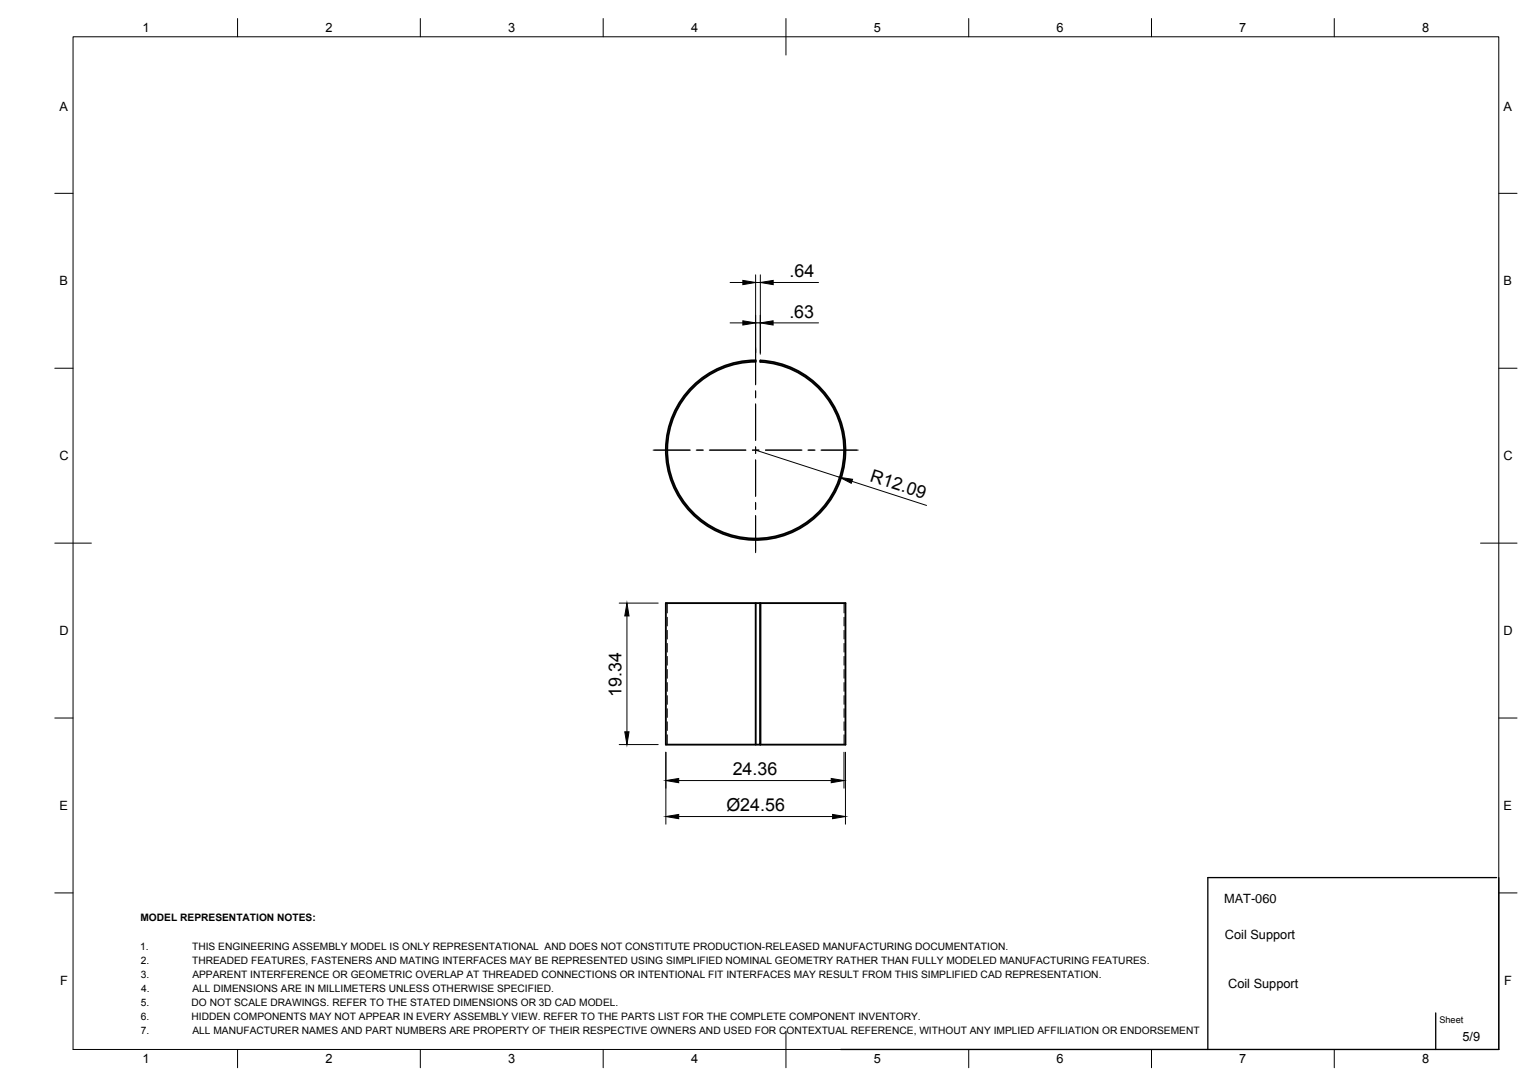
ISO-10303-21;
HEADER;
FILE_DESCRIPTION (('STEP AP214'),
    '1' );
FILE_NAME ('Coil Support.step',
    '2026-10-29T23:46:56',
    ( '' ),
    ( '' ),
    'SwSTEP 2.0',
    'SolidWorks 2020',
    '' );
FILE_SCHEMA (( 'AUTOMOTIVE_DESIGN' ));
ENDSEC;

DATA;
#93=APPLICATION_CONTEXT ( 'automotive_design' ) ;
#920=PLANE ( 'NONE',  #8989 ) ;
#938=UNCERTAINTY_MEASURE_WITH_UNIT (LENGTH_MEASURE( 1.000000000000000082E-05 ), #1682, 'distance_accuracy_value', 'NONE');
#1251=UNCERTAINTY_MEASURE_WITH_UNIT (LENGTH_MEASURE( 1.000000000000000082E-05 ), #14331, 'distance_accuracy_value', 'NONE');
#1354=DIRECTION ( 'NONE',  ( 0.000000000000000000, 0.000000000000000000, 1.000000000000000000 ) ) ;
#1682=( LENGTH_UNIT ( ) NAMED_UNIT ( * ) SI_UNIT ( .MILLI., .METRE. ) );
#1888=ADVANCED_FACE ( 'NONE', ( #14373 ), #14045, .F. ) ;
#2120=CIRCLE ( 'NONE', #12091, 12.08499999999999908 ) ;
#2336=DIRECTION ( 'NONE',  ( -1.000000000000000000, -6.722685822323786766E-17, 0.000000000000000000 ) ) ;
#2420=VECTOR ( 'NONE', #13652, 1000.000000000000000 ) ;
#2970=CARTESIAN_POINT ( 'NONE',  ( 8.823575513742490273, 15.24673779880127356, 47.37072134000479906 ) ) ;
#3223=FACE_OUTER_BOUND ( 'NONE', #6473, .T. ) ;
#3349=DIRECTION ( 'NONE',  ( -0.9996573249755574819, -1.344306794811909066E-16, 0.02617694830786587712 ) ) ;
#3732=ORIENTED_EDGE ( 'NONE', *, *, #20264, .T. ) ;
#3809=ADVANCED_FACE ( 'NONE', ( #18879 ), #11193, .T. ) ;
#3828=CARTESIAN_POINT ( 'NONE',  ( 8.823575513742486720, 34.59164230456639899, 47.37072134000479906 ) ) ;
#3965=EDGE_CURVE ( 'NONE', #14754, #4855, #5249, .T. ) ;
#4047=ORIENTED_EDGE ( 'NONE', *, *, #20264, .F. ) ;
#4080=CARTESIAN_POINT ( 'NONE',  ( 9.016997203727582288, 34.59164230456639899, 47.36565641480107303 ) ) ;
#4315=DIRECTION ( 'NONE',  ( -0.02617694830786587365, -1.759793992609925531E-18, 0.9996573249755574819 ) ) ;
#4409=ORIENTED_EDGE ( 'NONE', *, *, #26266, .F. ) ;
#4774=DIRECTION ( 'NONE',  ( -1.000000000000000000, 0.000000000000000000, 0.000000000000000000 ) ) ;
#4801=( NAMED_UNIT ( * ) SI_UNIT ( $, .STERADIAN. ) SOLID_ANGLE_UNIT ( ) );
#4810=CARTESIAN_POINT ( 'NONE',  ( 9.016997203727585841, 15.24673779880127356, 47.36565641480107303 ) ) ;
#4855=VERTEX_POINT ( 'NONE', #3828 ) ;
#4994=ORIENTED_EDGE ( 'NONE', *, *, #3965, .T. ) ;
#5249=LINE ( 'NONE', #15258, #5266 ) ;
#5266=VECTOR ( 'NONE', #25269, 1000.000000000000000 ) ;
#5378=CARTESIAN_POINT ( 'NONE',  ( 9.016997203727585841, 15.24673779880127356, 47.36565641480107303 ) ) ;
#5977=DIRECTION ( 'NONE',  ( 1.000000000000000000, 0.000000000000000000, 0.000000000000000000 ) ) ;
#6075=STYLED_ITEM ( 'NONE', ( #27283 ), #8502 ) ;
#6286=CARTESIAN_POINT ( 'NONE',  ( 0.000000000000000000, 0.000000000000000000, 0.000000000000000000 ) ) ;
#6354=ORIENTED_EDGE ( 'NONE', *, *, #20840, .T. ) ;
#6473=EDGE_LOOP ( 'NONE', ( #3732, #4994, #23188, #17455 ) ) ;
#6586=CARTESIAN_POINT ( 'NONE',  ( 21.09785597605719332, 34.59164230456639899, 47.04930799450051637 ) ) ;
#6613=( NAMED_UNIT ( * ) PLANE_ANGLE_UNIT ( ) SI_UNIT ( $, .RADIAN. ) );
#6740=VERTEX_POINT ( 'NONE', #4080 ) ;
#7156=PRODUCT_DEFINITION_CONTEXT ( 'detailed design', #29222, 'design' ) ;
#7164=ORIENTED_EDGE ( 'NONE', *, *, #11045, .F. ) ;
#7266=SURFACE_SIDE_STYLE ('',( #19066 ) ) ;
#7305=VERTEX_POINT ( 'NONE', #30199 ) ;
#8051=CARTESIAN_POINT ( 'NONE',  ( 9.016997203727585841, 15.24673779880127356, 46.73295957419995261 ) ) ;
#8162=DIRECTION ( 'NONE',  ( 0.02617694830786587712, 1.759793992609925531E-18, 0.9996573249755574819 ) ) ;
#8172=AXIS2_PLACEMENT_3D ( 'NONE', #6286, #1354, #5977 ) ;
#8284=CARTESIAN_POINT ( 'NONE',  ( 9.016997203727582288, 34.59164230456639899, 46.73295957419995261 ) ) ;
#8475=STYLED_ITEM('',(#32529),#12176);
#8502=ADVANCED_BREP_SHAPE_REPRESENTATION ( '', ( #12176, #8172 ), #26498 ) ;
#8989=AXIS2_PLACEMENT_3D ( 'NONE', #5378, #8162, #13260 ) ;
#9433=CARTESIAN_POINT ( 'NONE',  ( 8.823575513742490273, 15.24673779880127356, 47.37072134000479906 ) ) ;
#9482=ORIENTED_EDGE ( 'NONE', *, *, #11238, .T. ) ;
#9569=CARTESIAN_POINT ( 'NONE',  ( 9.016997203727585841, 15.24673779880127356, 46.73295957419995261 ) ) ;
#9604=ORIENTED_EDGE ( 'NONE', *, *, #19433, .F. ) ;
#9896=VECTOR ( 'NONE', #27905, 1000.000000000000000 ) ;
#10047=DIRECTION ( 'NONE',  ( -1.000000000000000000, 0.000000000000000000, 0.000000000000000000 ) ) ;
#10212=CARTESIAN_POINT ( 'NONE',  ( 9.016997203727582288, 34.59164230456639899, 46.73295957419995261 ) ) ;
#10249=ORIENTED_EDGE ( 'NONE', *, *, #26494, .F. ) ;
#10276=LINE ( 'NONE', #8284, #15201 ) ;
#10299=ORIENTED_EDGE ( 'NONE', *, *, #26494, .T. ) ;
#10924=CIRCLE ( 'NONE', #11970, 12.08499999999999552 ) ;
#11045=EDGE_CURVE ( 'NONE', #6740, #18267, #2120, .T. ) ;
#11193=CYLINDRICAL_SURFACE ( 'NONE', #18323, 12.27848799348799069 ) ;
#11238=EDGE_CURVE ( 'NONE', #14754, #7305, #26221, .T. ) ;
#11270=ORIENTED_EDGE ( 'NONE', *, *, #3965, .F. ) ;
#11397=CARTESIAN_POINT ( 'NONE',  ( 9.016997203727585841, 15.24673779880127356, 46.73295957419995261 ) ) ;
#11902=VECTOR ( 'NONE', #3349, 1000.000000000000000 ) ;
#11970=AXIS2_PLACEMENT_3D ( 'NONE', #15129, #20530, #10047 ) ;
#12091=AXIS2_PLACEMENT_3D ( 'NONE', #23892, #31452, #21581 ) ;
#12176=MANIFOLD_SOLID_BREP ( 'Stock-MAT-060-1', #23142 ) ;
#12366=MECHANICAL_DESIGN_GEOMETRIC_PRESENTATION_REPRESENTATION('',(#6075),#27557);
#12521=DIRECTION ( 'NONE',  ( -6.722685822323786766E-17, 1.000000000000000000, 0.000000000000000000 ) ) ;
#12678=AXIS2_PLACEMENT_3D ( 'NONE', #31928, #31606, #19108 ) ;
#12697=LINE ( 'NONE', #20218, #2420 ) ;
#13004=FACE_OUTER_BOUND ( 'NONE', #28868, .T. ) ;
#13260=DIRECTION ( 'NONE',  ( 0.9996573249755574819, 1.344306794811909066E-16, -0.02617694830786587712 ) ) ;
#13530=CARTESIAN_POINT ( 'NONE',  ( 8.823575513742490273, 15.24673779880127356, 47.37072134000479906 ) ) ;
#13602=ORIENTED_EDGE ( 'NONE', *, *, #19433, .T. ) ;
#13652=DIRECTION ( 'NONE',  ( -0.9996573249755574819, -1.344306794811909066E-16, -0.02617694830786587365 ) ) ;
#14019=VECTOR ( 'NONE', #17603, 1000.000000000000000 ) ;
#14045=PLANE ( 'NONE',  #12678 ) ;
#14211=ORIENTED_EDGE ( 'NONE', *, *, #11045, .T. ) ;
#14331=( LENGTH_UNIT ( ) NAMED_UNIT ( * ) SI_UNIT ( .MILLI., .METRE. ) );
#14373=FACE_OUTER_BOUND ( 'NONE', #16626, .T. ) ;
#14561=DIRECTION ( 'NONE',  ( -1.000000000000000000, 0.000000000000000000, 0.000000000000000000 ) ) ;
#14754=VERTEX_POINT ( 'NONE', #9433 ) ;
#14791=DIRECTION ( 'NONE',  ( -6.722685822323786766E-17, 1.000000000000000000, -0.000000000000000000 ) ) ;
#14818=PRODUCT_DEFINITION_SHAPE ( 'NONE', 'NONE',  #27968 ) ;
#15129=CARTESIAN_POINT ( 'NONE',  ( 21.09785597605719332, 15.24673779880127356, 47.04930799450051637 ) ) ;
#15201=VECTOR ( 'NONE', #18279, 1000.000000000000000 ) ;
#15258=CARTESIAN_POINT ( 'NONE',  ( 8.823575513742486720, 34.59164230456639899, 47.37072134000479906 ) ) ;
#15575=EDGE_LOOP ( 'NONE', ( #14211, #10299, #21457, #30476 ) ) ;
#16015=ORIENTED_EDGE ( 'NONE', *, *, #26379, .F. ) ;
#16268=AXIS2_PLACEMENT_3D ( 'NONE', #21683, #22417, #14561 ) ;
#16606=( NAMED_UNIT ( * ) SI_UNIT ( $, .STERADIAN. ) SOLID_ANGLE_UNIT ( ) );
#16626=EDGE_LOOP ( 'NONE', ( #6354, #29197, #7164, #16015 ) ) ;
#16731=LINE ( 'NONE', #21984, #26653 ) ;
#16988=UNCERTAINTY_MEASURE_WITH_UNIT (LENGTH_MEASURE( 1.000000000000000082E-05 ), #22510, 'distance_accuracy_value', 'NONE');
#17018=SHAPE_REPRESENTATION ( 'Coil Support', ( #8172 ), #26498 ) ;
#17107=DIRECTION ( 'NONE',  ( -1.000000000000000000, 0.000000000000000000, 0.000000000000000000 ) ) ;
#17455=ORIENTED_EDGE ( 'NONE', *, *, #20567, .T. ) ;
#17564=VERTEX_POINT ( 'NONE', #18098 ) ;
#17603=DIRECTION ( 'NONE',  ( 1.344306794811909313E-16, -1.000000000000000000, -1.759793992609926301E-18 ) ) ;
#17717=LINE ( 'NONE', #8051, #9896 ) ;
#17761=VECTOR ( 'NONE', #21172, 1000.000000000000000 ) ;
#18076=VERTEX_POINT ( 'NONE', #30601 ) ;
#18098=CARTESIAN_POINT ( 'NONE',  ( 8.823575513742486720, 34.59164230456639899, 46.72789464899623368 ) ) ;
#18231=CARTESIAN_POINT ( 'NONE',  ( 8.823575513742486720, 34.59164230456639899, 46.72789464899623368 ) ) ;
#18267=VERTEX_POINT ( 'NONE', #10212 ) ;
#18279=DIRECTION ( 'NONE',  ( 0.9996573249755574819, 1.344306794811909066E-16, 0.02617694830786587365 ) ) ;
#18323=AXIS2_PLACEMENT_3D ( 'NONE', #21176, #31219, #26599 ) ;
#18408=AXIS2_PLACEMENT_3D ( 'NONE', #2970, #12521, #2336 ) ;
#18879=FACE_OUTER_BOUND ( 'NONE', #20657, .T. ) ;
#19066=SURFACE_STYLE_FILL_AREA ( #31882 ) ;
#19108=DIRECTION ( 'NONE',  ( 1.000000000000000000, 6.722685822323786766E-17, 0.000000000000000000 ) ) ;
#19197=DIRECTION ( 'NONE',  ( 0.9996573249755574819, 1.344306794811909066E-16, -0.02617694830786587712 ) ) ;
#19226=( NAMED_UNIT ( * ) PLANE_ANGLE_UNIT ( ) SI_UNIT ( $, .RADIAN. ) );
#19433=EDGE_CURVE ( 'NONE', #22755, #7305, #12697, .T. ) ;
#19569=FACE_OUTER_BOUND ( 'NONE', #26876, .T. ) ;
#19779=PRODUCT ( 'Coil Support', 'Coil Support', '', ( #22958 ) ) ;
#19887=( NAMED_UNIT ( * ) SI_UNIT ( $, .STERADIAN. ) SOLID_ANGLE_UNIT ( ) );
#20019=SHAPE_DEFINITION_REPRESENTATION ( #14818, #17018 ) ;
#20218=CARTESIAN_POINT ( 'NONE',  ( 8.823575513742490273, 15.24673779880127356, 46.72789464899623368 ) ) ;
#20227=DIRECTION ( 'NONE',  ( -6.722685822323786766E-17, 1.000000000000000000, -0.000000000000000000 ) ) ;
#20264=EDGE_CURVE ( 'NONE', #18076, #14754, #31254, .T. ) ;
#20530=DIRECTION ( 'NONE',  ( -6.722685822323786766E-17, 1.000000000000000000, -0.000000000000000000 ) ) ;
#20567=EDGE_CURVE ( 'NONE', #6740, #18076, #27294, .T. ) ;
#20657=EDGE_LOOP ( 'NONE', ( #11270, #9482, #30639, #29511 ) ) ;
#20840=EDGE_CURVE ( 'NONE', #4855, #17564, #26607, .T. ) ;
#21172=DIRECTION ( 'NONE',  ( -1.344306794811909066E-16, 1.000000000000000000, -1.759793992609925531E-18 ) ) ;
#21176=CARTESIAN_POINT ( 'NONE',  ( 21.09785597605719332, 39.33406896771847983, 47.04930799450051637 ) ) ;
#21457=ORIENTED_EDGE ( 'NONE', *, *, #22818, .F. ) ;
#21581=DIRECTION ( 'NONE',  ( -1.000000000000000000, 0.000000000000000000, 0.000000000000000000 ) ) ;
#21683=CARTESIAN_POINT ( 'NONE',  ( 21.09785597605719332, 15.24673779880127356, 47.04930799450051637 ) ) ;
#21984=CARTESIAN_POINT ( 'NONE',  ( 9.016997203727582288, 34.59164230456639899, 47.36565641480107303 ) ) ;
#22122=AXIS2_PLACEMENT_3D ( 'NONE', #24837, #20227, #17107 ) ;
#22200=CYLINDRICAL_SURFACE ( 'NONE', #22122, 12.08499999999999730 ) ;
#22354=PLANE ( 'NONE',  #23506 ) ;
#22417=DIRECTION ( 'NONE',  ( -6.722685822323786766E-17, 1.000000000000000000, -0.000000000000000000 ) ) ;
#22510=( LENGTH_UNIT ( ) NAMED_UNIT ( * ) SI_UNIT ( .MILLI., .METRE. ) );
#22755=VERTEX_POINT ( 'NONE', #11397 ) ;
#22818=EDGE_CURVE ( 'NONE', #18076, #22755, #10924, .T. ) ;
#22864=ORIENTED_EDGE ( 'NONE', *, *, #22818, .T. ) ;
#22958=PRODUCT_CONTEXT ( 'NONE', #93, 'mechanical' ) ;
#23142=CLOSED_SHELL ( 'NONE', ( #25022, #30108, #1888, #3809, #25391, #26007 ) ) ;
#23188=ORIENTED_EDGE ( 'NONE', *, *, #26379, .T. ) ;
#23308=ORIENTED_EDGE ( 'NONE', *, *, #27010, .F. ) ;
#23506=AXIS2_PLACEMENT_3D ( 'NONE', #9569, #4315, #31886 ) ;
#23892=CARTESIAN_POINT ( 'NONE',  ( 21.09785597605719332, 34.59164230456639899, 47.04930799450051637 ) ) ;
#24518=AXIS2_PLACEMENT_3D ( 'NONE', #6586, #14791, #4774 ) ;
#24826=FILL_AREA_STYLE_COLOUR ( '', #31752 ) ;
#24837=CARTESIAN_POINT ( 'NONE',  ( 21.09785597605719332, 39.33406896771847983, 47.04930799450051637 ) ) ;
#25022=ADVANCED_FACE ( 'NONE', ( #13004 ), #30237, .F. ) ;
#25269=DIRECTION ( 'NONE',  ( -1.344306794811909313E-16, 1.000000000000000000, 1.759793992609926301E-18 ) ) ;
#25391=ADVANCED_FACE ( 'NONE', ( #3223 ), #920, .F. ) ;
#26007=ADVANCED_FACE ( 'NONE', ( #19569 ), #22354, .T. ) ;
#26221=CIRCLE ( 'NONE', #16268, 12.27848799348798892 ) ;
#26266=EDGE_CURVE ( 'NONE', #7305, #17564, #31369, .T. ) ;
#26379=EDGE_CURVE ( 'NONE', #4855, #6740, #16731, .T. ) ;
#26494=EDGE_CURVE ( 'NONE', #18267, #22755, #17717, .T. ) ;
#26498=( GEOMETRIC_REPRESENTATION_CONTEXT ( 3 ) GLOBAL_UNCERTAINTY_ASSIGNED_CONTEXT ( ( #1251 ) ) GLOBAL_UNIT_ASSIGNED_CONTEXT ( ( #14331, #19226, #4801 ) ) REPRESENTATION_CONTEXT ( 'NONE', 'WORKASPACE' ) );
#26599=DIRECTION ( 'NONE',  ( -1.000000000000000000, 0.000000000000000000, 0.000000000000000000 ) ) ;
#26607=CIRCLE ( 'NONE', #24518, 12.27848799348799069 ) ;
#26653=VECTOR ( 'NONE', #19197, 1000.000000000000000 ) ;
#26876=EDGE_LOOP ( 'NONE', ( #9604, #10249, #23308, #4409 ) ) ;
#27010=EDGE_CURVE ( 'NONE', #17564, #18267, #10276, .T. ) ;
#27283=PRESENTATION_STYLE_ASSIGNMENT (( #29098 ) ) ;
#27294=LINE ( 'NONE', #4810, #14019 ) ;
#27557=( GEOMETRIC_REPRESENTATION_CONTEXT ( 3 ) GLOBAL_UNCERTAINTY_ASSIGNED_CONTEXT ( ( #938 ) ) GLOBAL_UNIT_ASSIGNED_CONTEXT ( ( #1682, #6613, #16606 ) ) REPRESENTATION_CONTEXT ( 'NONE', 'WORKASPACE' ) );
#27905=DIRECTION ( 'NONE',  ( 1.344306794811909066E-16, -1.000000000000000000, 1.759793992609925531E-18 ) ) ;
#27968=PRODUCT_DEFINITION ( 'UNKNOWN', '', #31785, #7156 ) ;
#28868=EDGE_LOOP ( 'NONE', ( #22864, #13602, #29034, #4047 ) ) ;
#29034=ORIENTED_EDGE ( 'NONE', *, *, #11238, .F. ) ;
#29098=SURFACE_STYLE_USAGE ( .BOTH. , #7266 ) ;
#29197=ORIENTED_EDGE ( 'NONE', *, *, #27010, .T. ) ;
#29222=APPLICATION_CONTEXT ( 'automotive_design' ) ;
#29426=SHAPE_REPRESENTATION_RELATIONSHIP ( 'NONE' , 'NONE' ,  #17018, #8502 ) ;
#29451=( GEOMETRIC_REPRESENTATION_CONTEXT ( 3 ) GLOBAL_UNCERTAINTY_ASSIGNED_CONTEXT ( ( #16988 ) ) GLOBAL_UNIT_ASSIGNED_CONTEXT ( ( #22510, #31881, #19887 ) ) REPRESENTATION_CONTEXT ( 'NONE', 'WORKASPACE' ) );
#29511=ORIENTED_EDGE ( 'NONE', *, *, #20840, .F. ) ;
#29597=FACE_OUTER_BOUND ( 'NONE', #15575, .T. ) ;
#30108=ADVANCED_FACE ( 'NONE', ( #29597 ), #22200, .F. ) ;
#30199=CARTESIAN_POINT ( 'NONE',  ( 8.823575513742490273, 15.24673779880127356, 46.72789464899623368 ) ) ;
#30237=PLANE ( 'NONE',  #18408 ) ;
#30476=ORIENTED_EDGE ( 'NONE', *, *, #20567, .F. ) ;
#30601=CARTESIAN_POINT ( 'NONE',  ( 9.016997203727585841, 15.24673779880127356, 47.36565641480107303 ) ) ;
#30639=ORIENTED_EDGE ( 'NONE', *, *, #26266, .T. ) ;
#31219=DIRECTION ( 'NONE',  ( -6.722685822323786766E-17, 1.000000000000000000, -0.000000000000000000 ) ) ;
#31254=LINE ( 'NONE', #13530, #11902 ) ;
#31369=LINE ( 'NONE', #18231, #17761 ) ;
#31452=DIRECTION ( 'NONE',  ( -6.722685822323786766E-17, 1.000000000000000000, -0.000000000000000000 ) ) ;
#31606=DIRECTION ( 'NONE',  ( 6.722685822323786766E-17, -1.000000000000000000, 0.000000000000000000 ) ) ;
#31752=COLOUR_RGB ( '',0.7921568627450980005, 0.8196078431372548767, 0.9333333333333333481 ) ;
#31785=PRODUCT_DEFINITION_FORMATION_WITH_SPECIFIED_SOURCE ( 'ANY', '', #19779, .NOT_KNOWN. ) ;
#31881=( NAMED_UNIT ( * ) PLANE_ANGLE_UNIT ( ) SI_UNIT ( $, .RADIAN. ) );
#31882=FILL_AREA_STYLE ('',( #24826 ) ) ;
#31886=DIRECTION ( 'NONE',  ( 0.9996573249755574819, 1.344306794811909066E-16, 0.02617694830786587365 ) ) ;
#31928=CARTESIAN_POINT ( 'NONE',  ( 9.016997203727582288, 34.59164230456639899, 47.36565641480107303 ) ) ;
#32075=MECHANICAL_DESIGN_GEOMETRIC_PRESENTATION_REPRESENTATION('',(#8475),#29451);
#32523=COLOUR_RGB('Sky Blue',0.24,0.69,0.87);
#32524=FILL_AREA_STYLE_COLOUR('',#32523);
#32525=FILL_AREA_STYLE('',(#32524));
#32526=SURFACE_STYLE_FILL_AREA(#32525);
#32527=SURFACE_SIDE_STYLE('',(#32526));
#32528=SURFACE_STYLE_USAGE(.BOTH.,#32527);
#32529=PRESENTATION_STYLE_ASSIGNMENT((#32528));
ENDSEC;
END-ISO-10303-21;
